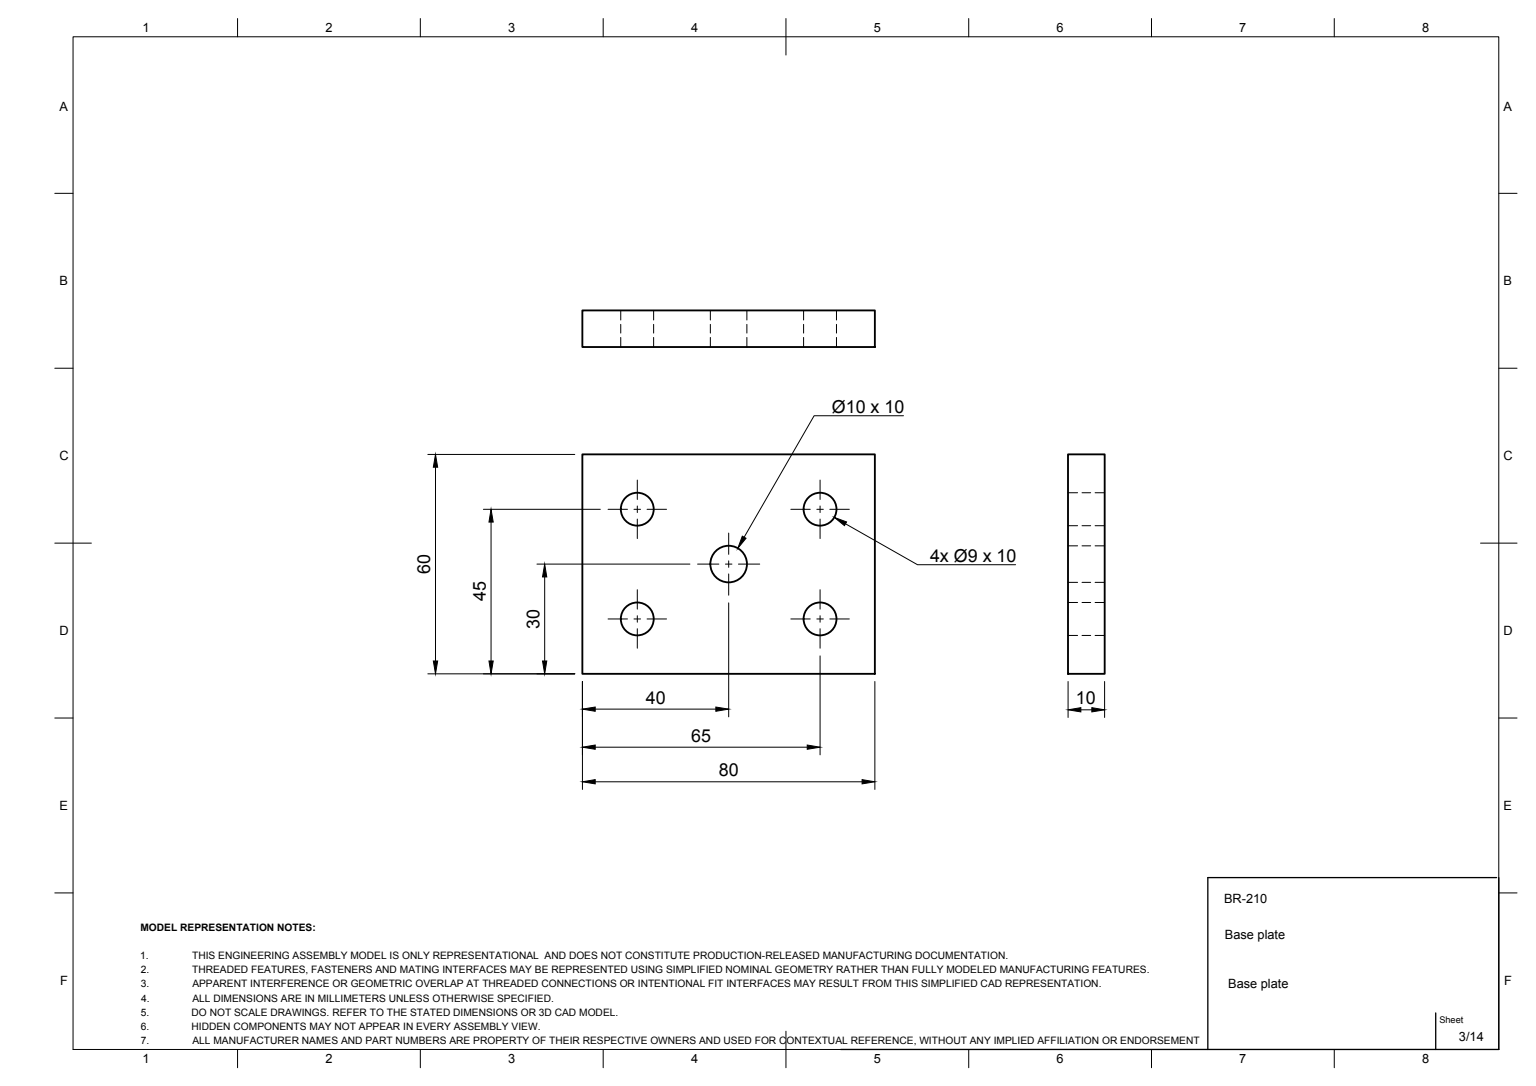
ISO-10303-21;
HEADER;
/* Generated by software containing ST-Developer
 * from STEP Tools, Inc. (www.steptools.com) 
 */

FILE_DESCRIPTION(
/* description */ ('Independent 1:2 reduction pantograph. 120 mm parallelogram sides; fix
ed fulcrum on the extension of a 240 mm link. Drawing point halfway al
ong its link, so its XY displacement is one half of the tracing point.
 Replaceable pivot bushes and retained pins. Calibration and productio
n accuracy unassigned.'),
/* implementation_level */ '2;1');

FILE_NAME(
/* name */ 'Base plate.step',
/* time_stamp */ '2026-11-07T22:11:57-08:00',
/* author */ (''),
/* organization */ (''),
/* preprocessor_version */ 'ST-DEVELOPER v20.2',
/* originating_system */ 'Autodesk Translation Framework v15.17.0.0',
/* authorisation */ '');

FILE_SCHEMA (('AUTOMOTIVE_DESIGN { 1 0 10303 214 3 1 1 }'));
ENDSEC;

DATA;
#10=MECHANICAL_DESIGN_GEOMETRIC_PRESENTATION_REPRESENTATION('',(#186),#2926);
#160=SHAPE_REPRESENTATION_RELATIONSHIP('SRR','None',#2997,#173);
#173=ADVANCED_BREP_SHAPE_REPRESENTATION('',(#199),#2913);
#186=STYLED_ITEM('',(#3071),#199);
#199=MANIFOLD_SOLID_BREP('Body1',#1541);
#212=FACE_BOUND('',#407,.T.);
#213=FACE_BOUND('',#408,.T.);
#214=FACE_BOUND('',#409,.T.);
#215=FACE_BOUND('',#410,.T.);
#216=FACE_BOUND('',#411,.T.);
#217=FACE_BOUND('',#413,.T.);
#218=FACE_BOUND('',#414,.T.);
#219=FACE_BOUND('',#415,.T.);
#220=FACE_BOUND('',#416,.T.);
#221=FACE_BOUND('',#417,.T.);
#258=PLANE('',#1715);
#259=PLANE('',#1716);
#260=PLANE('',#1717);
#261=PLANE('',#1718);
#262=PLANE('',#1719);
#263=PLANE('',#1720);
#305=FACE_OUTER_BOUND('',#397,.T.);
#306=FACE_OUTER_BOUND('',#398,.T.);
#307=FACE_OUTER_BOUND('',#399,.T.);
#308=FACE_OUTER_BOUND('',#400,.T.);
#309=FACE_OUTER_BOUND('',#401,.T.);
#310=FACE_OUTER_BOUND('',#402,.T.);
#311=FACE_OUTER_BOUND('',#403,.T.);
#312=FACE_OUTER_BOUND('',#404,.T.);
#313=FACE_OUTER_BOUND('',#405,.T.);
#314=FACE_OUTER_BOUND('',#406,.T.);
#315=FACE_OUTER_BOUND('',#412,.T.);
#397=EDGE_LOOP('',(#1067,#1068,#1069,#1070));
#398=EDGE_LOOP('',(#1071,#1072,#1073,#1074));
#399=EDGE_LOOP('',(#1075,#1076,#1077,#1078));
#400=EDGE_LOOP('',(#1079,#1080,#1081,#1082));
#401=EDGE_LOOP('',(#1083,#1084,#1085,#1086));
#402=EDGE_LOOP('',(#1087,#1088,#1089,#1090));
#403=EDGE_LOOP('',(#1091,#1092,#1093,#1094));
#404=EDGE_LOOP('',(#1095,#1096,#1097,#1098));
#405=EDGE_LOOP('',(#1099,#1100,#1101,#1102));
#406=EDGE_LOOP('',(#1103,#1104,#1105,#1106));
#407=EDGE_LOOP('',(#1107));
#408=EDGE_LOOP('',(#1108));
#409=EDGE_LOOP('',(#1109));
#410=EDGE_LOOP('',(#1110));
#411=EDGE_LOOP('',(#1111));
#412=EDGE_LOOP('',(#1112,#1113,#1114,#1115));
#413=EDGE_LOOP('',(#1116));
#414=EDGE_LOOP('',(#1117));
#415=EDGE_LOOP('',(#1118));
#416=EDGE_LOOP('',(#1119));
#417=EDGE_LOOP('',(#1120));
#535=LINE('',#2478,#616);
#536=LINE('',#2484,#617);
#537=LINE('',#2490,#618);
#538=LINE('',#2496,#619);
#539=LINE('',#2502,#620);
#540=LINE('',#2507,#621);
#541=LINE('',#2509,#622);
#542=LINE('',#2511,#623);
#543=LINE('',#2512,#624);
#544=LINE('',#2515,#625);
#545=LINE('',#2517,#626);
#546=LINE('',#2518,#627);
#547=LINE('',#2521,#628);
#548=LINE('',#2523,#629);
#549=LINE('',#2524,#630);
#550=LINE('',#2526,#631);
#551=LINE('',#2527,#632);
#616=VECTOR('',#1937,4.5);
#617=VECTOR('',#1944,4.5);
#618=VECTOR('',#1951,4.5);
#619=VECTOR('',#1958,4.5);
#620=VECTOR('',#1965,5.);
#621=VECTOR('',#1970,10.);
#622=VECTOR('',#1971,10.);
#623=VECTOR('',#1972,10.);
#624=VECTOR('',#1973,10.);
#625=VECTOR('',#1976,10.);
#626=VECTOR('',#1977,10.);
#627=VECTOR('',#1978,10.);
#628=VECTOR('',#1981,10.);
#629=VECTOR('',#1982,10.);
#630=VECTOR('',#1983,10.);
#631=VECTOR('',#1986,10.);
#632=VECTOR('',#1987,10.);
#697=CIRCLE('',#1701,4.5);
#698=CIRCLE('',#1702,4.5);
#699=CIRCLE('',#1704,4.5);
#700=CIRCLE('',#1705,4.5);
#701=CIRCLE('',#1707,4.5);
#702=CIRCLE('',#1708,4.5);
#703=CIRCLE('',#1710,4.5);
#704=CIRCLE('',#1711,4.5);
#705=CIRCLE('',#1713,5.);
#706=CIRCLE('',#1714,5.);
#785=VERTEX_POINT('',#2475);
#786=VERTEX_POINT('',#2477);
#787=VERTEX_POINT('',#2481);
#788=VERTEX_POINT('',#2483);
#789=VERTEX_POINT('',#2487);
#790=VERTEX_POINT('',#2489);
#791=VERTEX_POINT('',#2493);
#792=VERTEX_POINT('',#2495);
#793=VERTEX_POINT('',#2499);
#794=VERTEX_POINT('',#2501);
#795=VERTEX_POINT('',#2505);
#796=VERTEX_POINT('',#2506);
#797=VERTEX_POINT('',#2508);
#798=VERTEX_POINT('',#2510);
#799=VERTEX_POINT('',#2514);
#800=VERTEX_POINT('',#2516);
#801=VERTEX_POINT('',#2520);
#802=VERTEX_POINT('',#2522);
#898=EDGE_CURVE('',#785,#785,#697,.T.);
#899=EDGE_CURVE('',#785,#786,#535,.T.);
#900=EDGE_CURVE('',#786,#786,#698,.T.);
#901=EDGE_CURVE('',#787,#787,#699,.T.);
#902=EDGE_CURVE('',#787,#788,#536,.T.);
#903=EDGE_CURVE('',#788,#788,#700,.T.);
#904=EDGE_CURVE('',#789,#789,#701,.T.);
#905=EDGE_CURVE('',#789,#790,#537,.T.);
#906=EDGE_CURVE('',#790,#790,#702,.T.);
#907=EDGE_CURVE('',#791,#791,#703,.T.);
#908=EDGE_CURVE('',#791,#792,#538,.T.);
#909=EDGE_CURVE('',#792,#792,#704,.T.);
#910=EDGE_CURVE('',#793,#793,#705,.T.);
#911=EDGE_CURVE('',#793,#794,#539,.T.);
#912=EDGE_CURVE('',#794,#794,#706,.T.);
#913=EDGE_CURVE('',#795,#796,#540,.T.);
#914=EDGE_CURVE('',#796,#797,#541,.T.);
#915=EDGE_CURVE('',#798,#797,#542,.T.);
#916=EDGE_CURVE('',#795,#798,#543,.T.);
#917=EDGE_CURVE('',#799,#795,#544,.T.);
#918=EDGE_CURVE('',#800,#798,#545,.T.);
#919=EDGE_CURVE('',#799,#800,#546,.T.);
#920=EDGE_CURVE('',#801,#799,#547,.T.);
#921=EDGE_CURVE('',#802,#800,#548,.T.);
#922=EDGE_CURVE('',#801,#802,#549,.T.);
#923=EDGE_CURVE('',#796,#801,#550,.T.);
#924=EDGE_CURVE('',#797,#802,#551,.T.);
#1067=ORIENTED_EDGE('',*,*,#898,.F.);
#1068=ORIENTED_EDGE('',*,*,#899,.T.);
#1069=ORIENTED_EDGE('',*,*,#900,.F.);
#1070=ORIENTED_EDGE('',*,*,#899,.F.);
#1071=ORIENTED_EDGE('',*,*,#901,.F.);
#1072=ORIENTED_EDGE('',*,*,#902,.T.);
#1073=ORIENTED_EDGE('',*,*,#903,.F.);
#1074=ORIENTED_EDGE('',*,*,#902,.F.);
#1075=ORIENTED_EDGE('',*,*,#904,.F.);
#1076=ORIENTED_EDGE('',*,*,#905,.T.);
#1077=ORIENTED_EDGE('',*,*,#906,.F.);
#1078=ORIENTED_EDGE('',*,*,#905,.F.);
#1079=ORIENTED_EDGE('',*,*,#907,.F.);
#1080=ORIENTED_EDGE('',*,*,#908,.T.);
#1081=ORIENTED_EDGE('',*,*,#909,.F.);
#1082=ORIENTED_EDGE('',*,*,#908,.F.);
#1083=ORIENTED_EDGE('',*,*,#910,.F.);
#1084=ORIENTED_EDGE('',*,*,#911,.T.);
#1085=ORIENTED_EDGE('',*,*,#912,.F.);
#1086=ORIENTED_EDGE('',*,*,#911,.F.);
#1087=ORIENTED_EDGE('',*,*,#913,.T.);
#1088=ORIENTED_EDGE('',*,*,#914,.T.);
#1089=ORIENTED_EDGE('',*,*,#915,.F.);
#1090=ORIENTED_EDGE('',*,*,#916,.F.);
#1091=ORIENTED_EDGE('',*,*,#917,.T.);
#1092=ORIENTED_EDGE('',*,*,#916,.T.);
#1093=ORIENTED_EDGE('',*,*,#918,.F.);
#1094=ORIENTED_EDGE('',*,*,#919,.F.);
#1095=ORIENTED_EDGE('',*,*,#920,.T.);
#1096=ORIENTED_EDGE('',*,*,#919,.T.);
#1097=ORIENTED_EDGE('',*,*,#921,.F.);
#1098=ORIENTED_EDGE('',*,*,#922,.F.);
#1099=ORIENTED_EDGE('',*,*,#923,.T.);
#1100=ORIENTED_EDGE('',*,*,#922,.T.);
#1101=ORIENTED_EDGE('',*,*,#924,.F.);
#1102=ORIENTED_EDGE('',*,*,#914,.F.);
#1103=ORIENTED_EDGE('',*,*,#924,.T.);
#1104=ORIENTED_EDGE('',*,*,#921,.T.);
#1105=ORIENTED_EDGE('',*,*,#918,.T.);
#1106=ORIENTED_EDGE('',*,*,#915,.T.);
#1107=ORIENTED_EDGE('',*,*,#910,.T.);
#1108=ORIENTED_EDGE('',*,*,#907,.T.);
#1109=ORIENTED_EDGE('',*,*,#904,.T.);
#1110=ORIENTED_EDGE('',*,*,#901,.T.);
#1111=ORIENTED_EDGE('',*,*,#898,.T.);
#1112=ORIENTED_EDGE('',*,*,#923,.F.);
#1113=ORIENTED_EDGE('',*,*,#913,.F.);
#1114=ORIENTED_EDGE('',*,*,#917,.F.);
#1115=ORIENTED_EDGE('',*,*,#920,.F.);
#1116=ORIENTED_EDGE('',*,*,#912,.T.);
#1117=ORIENTED_EDGE('',*,*,#909,.T.);
#1118=ORIENTED_EDGE('',*,*,#906,.T.);
#1119=ORIENTED_EDGE('',*,*,#903,.T.);
#1120=ORIENTED_EDGE('',*,*,#900,.T.);
#1405=CYLINDRICAL_SURFACE('',#1700,4.5);
#1406=CYLINDRICAL_SURFACE('',#1703,4.5);
#1407=CYLINDRICAL_SURFACE('',#1706,4.5);
#1408=CYLINDRICAL_SURFACE('',#1709,4.5);
#1409=CYLINDRICAL_SURFACE('',#1712,5.);
#1449=ADVANCED_FACE('',(#305),#1405,.F.);
#1450=ADVANCED_FACE('',(#306),#1406,.F.);
#1451=ADVANCED_FACE('',(#307),#1407,.F.);
#1452=ADVANCED_FACE('',(#308),#1408,.F.);
#1453=ADVANCED_FACE('',(#309),#1409,.F.);
#1454=ADVANCED_FACE('',(#310),#258,.T.);
#1455=ADVANCED_FACE('',(#311),#259,.T.);
#1456=ADVANCED_FACE('',(#312),#260,.T.);
#1457=ADVANCED_FACE('',(#313),#261,.T.);
#1458=ADVANCED_FACE('',(#314,#212,#213,#214,#215,#216),#262,.T.);
#1459=ADVANCED_FACE('',(#315,#217,#218,#219,#220,#221),#263,.F.);
#1541=CLOSED_SHELL('',(#1449,#1450,#1451,#1452,#1453,#1454,#1455,#1456,
#1457,#1458,#1459));
#1699=AXIS2_PLACEMENT_3D('',#2473,#1931,#1932);
#1700=AXIS2_PLACEMENT_3D('',#2474,#1933,#1934);
#1701=AXIS2_PLACEMENT_3D('',#2476,#1935,#1936);
#1702=AXIS2_PLACEMENT_3D('',#2479,#1938,#1939);
#1703=AXIS2_PLACEMENT_3D('',#2480,#1940,#1941);
#1704=AXIS2_PLACEMENT_3D('',#2482,#1942,#1943);
#1705=AXIS2_PLACEMENT_3D('',#2485,#1945,#1946);
#1706=AXIS2_PLACEMENT_3D('',#2486,#1947,#1948);
#1707=AXIS2_PLACEMENT_3D('',#2488,#1949,#1950);
#1708=AXIS2_PLACEMENT_3D('',#2491,#1952,#1953);
#1709=AXIS2_PLACEMENT_3D('',#2492,#1954,#1955);
#1710=AXIS2_PLACEMENT_3D('',#2494,#1956,#1957);
#1711=AXIS2_PLACEMENT_3D('',#2497,#1959,#1960);
#1712=AXIS2_PLACEMENT_3D('',#2498,#1961,#1962);
#1713=AXIS2_PLACEMENT_3D('',#2500,#1963,#1964);
#1714=AXIS2_PLACEMENT_3D('',#2503,#1966,#1967);
#1715=AXIS2_PLACEMENT_3D('',#2504,#1968,#1969);
#1716=AXIS2_PLACEMENT_3D('',#2513,#1974,#1975);
#1717=AXIS2_PLACEMENT_3D('',#2519,#1979,#1980);
#1718=AXIS2_PLACEMENT_3D('',#2525,#1984,#1985);
#1719=AXIS2_PLACEMENT_3D('',#2528,#1988,#1989);
#1720=AXIS2_PLACEMENT_3D('',#2529,#1990,#1991);
#1931=DIRECTION('axis',(0.,0.,1.));
#1932=DIRECTION('refdir',(1.,0.,0.));
#1933=DIRECTION('center_axis',(0.,0.,-1.));
#1934=DIRECTION('ref_axis',(1.,0.,0.));
#1935=DIRECTION('center_axis',(0.,0.,-1.));
#1936=DIRECTION('ref_axis',(1.,0.,0.));
#1937=DIRECTION('',(0.,0.,-1.));
#1938=DIRECTION('center_axis',(0.,0.,1.));
#1939=DIRECTION('ref_axis',(1.,0.,0.));
#1940=DIRECTION('center_axis',(0.,0.,-1.));
#1941=DIRECTION('ref_axis',(1.,0.,0.));
#1942=DIRECTION('center_axis',(0.,0.,-1.));
#1943=DIRECTION('ref_axis',(1.,0.,0.));
#1944=DIRECTION('',(0.,0.,-1.));
#1945=DIRECTION('center_axis',(0.,0.,1.));
#1946=DIRECTION('ref_axis',(1.,0.,0.));
#1947=DIRECTION('center_axis',(0.,0.,-1.));
#1948=DIRECTION('ref_axis',(1.,0.,0.));
#1949=DIRECTION('center_axis',(0.,0.,-1.));
#1950=DIRECTION('ref_axis',(1.,0.,0.));
#1951=DIRECTION('',(0.,0.,-1.));
#1952=DIRECTION('center_axis',(0.,0.,1.));
#1953=DIRECTION('ref_axis',(1.,0.,0.));
#1954=DIRECTION('center_axis',(0.,0.,-1.));
#1955=DIRECTION('ref_axis',(1.,0.,0.));
#1956=DIRECTION('center_axis',(0.,0.,-1.));
#1957=DIRECTION('ref_axis',(1.,0.,0.));
#1958=DIRECTION('',(0.,0.,-1.));
#1959=DIRECTION('center_axis',(0.,0.,1.));
#1960=DIRECTION('ref_axis',(1.,0.,0.));
#1961=DIRECTION('center_axis',(0.,0.,-1.));
#1962=DIRECTION('ref_axis',(1.,0.,0.));
#1963=DIRECTION('center_axis',(0.,0.,-1.));
#1964=DIRECTION('ref_axis',(1.,0.,0.));
#1965=DIRECTION('',(0.,0.,-1.));
#1966=DIRECTION('center_axis',(0.,0.,1.));
#1967=DIRECTION('ref_axis',(1.,0.,0.));
#1968=DIRECTION('center_axis',(0.,1.,0.));
#1969=DIRECTION('ref_axis',(-1.,0.,0.));
#1970=DIRECTION('',(-1.,0.,0.));
#1971=DIRECTION('',(0.,0.,1.));
#1972=DIRECTION('',(-1.,0.,0.));
#1973=DIRECTION('',(0.,0.,1.));
#1974=DIRECTION('center_axis',(1.,0.,0.));
#1975=DIRECTION('ref_axis',(0.,1.,0.));
#1976=DIRECTION('',(0.,1.,0.));
#1977=DIRECTION('',(0.,1.,0.));
#1978=DIRECTION('',(0.,0.,1.));
#1979=DIRECTION('center_axis',(0.,-1.,0.));
#1980=DIRECTION('ref_axis',(1.,0.,0.));
#1981=DIRECTION('',(1.,0.,0.));
#1982=DIRECTION('',(1.,0.,0.));
#1983=DIRECTION('',(0.,0.,1.));
#1984=DIRECTION('center_axis',(-1.,0.,0.));
#1985=DIRECTION('ref_axis',(0.,-1.,0.));
#1986=DIRECTION('',(0.,-1.,0.));
#1987=DIRECTION('',(0.,-1.,0.));
#1988=DIRECTION('center_axis',(0.,0.,1.));
#1989=DIRECTION('ref_axis',(1.,0.,0.));
#1990=DIRECTION('center_axis',(0.,0.,1.));
#1991=DIRECTION('ref_axis',(1.,0.,0.));
#2473=CARTESIAN_POINT('',(0.,0.,0.));
#2474=CARTESIAN_POINT('Origin',(25.,-15.,5.));
#2475=CARTESIAN_POINT('',(20.5,-15.,10.));
#2476=CARTESIAN_POINT('Origin',(25.,-15.,10.));
#2477=CARTESIAN_POINT('',(20.5,-15.,0.));
#2478=CARTESIAN_POINT('',(20.5,-15.,5.));
#2479=CARTESIAN_POINT('Origin',(25.,-15.,0.));
#2480=CARTESIAN_POINT('Origin',(-25.,-15.,5.));
#2481=CARTESIAN_POINT('',(-29.5,-15.,10.));
#2482=CARTESIAN_POINT('Origin',(-25.,-15.,10.));
#2483=CARTESIAN_POINT('',(-29.5,-15.,0.));
#2484=CARTESIAN_POINT('',(-29.5,-15.,5.));
#2485=CARTESIAN_POINT('Origin',(-25.,-15.,0.));
#2486=CARTESIAN_POINT('Origin',(-25.,15.,5.));
#2487=CARTESIAN_POINT('',(-29.5,15.,10.));
#2488=CARTESIAN_POINT('Origin',(-25.,15.,10.));
#2489=CARTESIAN_POINT('',(-29.5,15.,0.));
#2490=CARTESIAN_POINT('',(-29.5,15.,5.));
#2491=CARTESIAN_POINT('Origin',(-25.,15.,0.));
#2492=CARTESIAN_POINT('Origin',(25.,15.,5.));
#2493=CARTESIAN_POINT('',(20.5,15.,10.));
#2494=CARTESIAN_POINT('Origin',(25.,15.,10.));
#2495=CARTESIAN_POINT('',(20.5,15.,0.));
#2496=CARTESIAN_POINT('',(20.5,15.,5.));
#2497=CARTESIAN_POINT('Origin',(25.,15.,0.));
#2498=CARTESIAN_POINT('Origin',(0.,0.,5.));
#2499=CARTESIAN_POINT('',(-5.,6.12323399573677E-16,10.));
#2500=CARTESIAN_POINT('Origin',(0.,0.,10.));
#2501=CARTESIAN_POINT('',(-5.,6.12323399573677E-16,0.));
#2502=CARTESIAN_POINT('',(-5.,6.12323399573677E-16,5.));
#2503=CARTESIAN_POINT('Origin',(0.,0.,0.));
#2504=CARTESIAN_POINT('Origin',(40.,30.,0.));
#2505=CARTESIAN_POINT('',(40.,30.,0.));
#2506=CARTESIAN_POINT('',(-40.,30.,0.));
#2507=CARTESIAN_POINT('',(40.,30.,0.));
#2508=CARTESIAN_POINT('',(-40.,30.,10.));
#2509=CARTESIAN_POINT('',(-40.,30.,0.));
#2510=CARTESIAN_POINT('',(40.,30.,10.));
#2511=CARTESIAN_POINT('',(40.,30.,10.));
#2512=CARTESIAN_POINT('',(40.,30.,0.));
#2513=CARTESIAN_POINT('Origin',(40.,-30.,0.));
#2514=CARTESIAN_POINT('',(40.,-30.,0.));
#2515=CARTESIAN_POINT('',(40.,-30.,0.));
#2516=CARTESIAN_POINT('',(40.,-30.,10.));
#2517=CARTESIAN_POINT('',(40.,-30.,10.));
#2518=CARTESIAN_POINT('',(40.,-30.,0.));
#2519=CARTESIAN_POINT('Origin',(-40.,-30.,0.));
#2520=CARTESIAN_POINT('',(-40.,-30.,0.));
#2521=CARTESIAN_POINT('',(-40.,-30.,0.));
#2522=CARTESIAN_POINT('',(-40.,-30.,10.));
#2523=CARTESIAN_POINT('',(-40.,-30.,10.));
#2524=CARTESIAN_POINT('',(-40.,-30.,0.));
#2525=CARTESIAN_POINT('Origin',(-40.,30.,0.));
#2526=CARTESIAN_POINT('',(-40.,30.,0.));
#2527=CARTESIAN_POINT('',(-40.,30.,10.));
#2528=CARTESIAN_POINT('Origin',(0.,0.,10.));
#2529=CARTESIAN_POINT('Origin',(0.,0.,0.));
#2898=UNCERTAINTY_MEASURE_WITH_UNIT(LENGTH_MEASURE(0.01),#2927,
'DISTANCE_ACCURACY_VALUE',
'Maximum model space distance between geometric entities at asserted c
onnectivities');
#2911=UNCERTAINTY_MEASURE_WITH_UNIT(LENGTH_MEASURE(0.01),#2927,
'DISTANCE_ACCURACY_VALUE',
'Maximum model space distance between geometric entities at asserted c
onnectivities');
#2913=(
GEOMETRIC_REPRESENTATION_CONTEXT(3)
GLOBAL_UNCERTAINTY_ASSIGNED_CONTEXT((#2898))
GLOBAL_UNIT_ASSIGNED_CONTEXT((#2927,#2929,#2930))
REPRESENTATION_CONTEXT('','3D')
);
#2926=(
GEOMETRIC_REPRESENTATION_CONTEXT(3)
GLOBAL_UNCERTAINTY_ASSIGNED_CONTEXT((#2911))
GLOBAL_UNIT_ASSIGNED_CONTEXT((#2927,#2929,#2930))
REPRESENTATION_CONTEXT('','3D')
);
#2927=(
LENGTH_UNIT()
NAMED_UNIT(*)
SI_UNIT(.MILLI.,.METRE.)
);
#2929=(
NAMED_UNIT(*)
PLANE_ANGLE_UNIT()
SI_UNIT($,.RADIAN.)
);
#2930=(
NAMED_UNIT(*)
SI_UNIT($,.STERADIAN.)
SOLID_ANGLE_UNIT()
);
#2932=SHAPE_DEFINITION_REPRESENTATION(#2946,#2997);
#2946=PRODUCT_DEFINITION_SHAPE('',$,#3012);
#2997=SHAPE_REPRESENTATION('',(#1699),#2913);
#3010=PRODUCT_DEFINITION_CONTEXT('part definition',#3054,'design');
#3012=PRODUCT_DEFINITION('Base plate','Base plate',#3026,#3010);
#3026=PRODUCT_DEFINITION_FORMATION('',$,#3057);
#3054=APPLICATION_CONTEXT(
'Core Data for Automotive Mechanical Design Process');
#3055=PRODUCT_CONTEXT('part definition',#3054,'mechanical');
#3057=PRODUCT('Base plate','Base plate','Base plate',(#3055));
#3071=PRESENTATION_STYLE_ASSIGNMENT((#3083));
#3083=SURFACE_STYLE_USAGE(.BOTH.,#3095);
#3095=SURFACE_SIDE_STYLE('',(#3107));
#3107=SURFACE_STYLE_FILL_AREA(#3119);
#3119=FILL_AREA_STYLE('Base gray',(#3131));
#3131=FILL_AREA_STYLE_COLOUR('Base gray',#3143);
#3143=COLOUR_RGB('Base gray',0.407843137254902,0.447058823529412,0.498039215686275);
ENDSEC;
END-ISO-10303-21;
